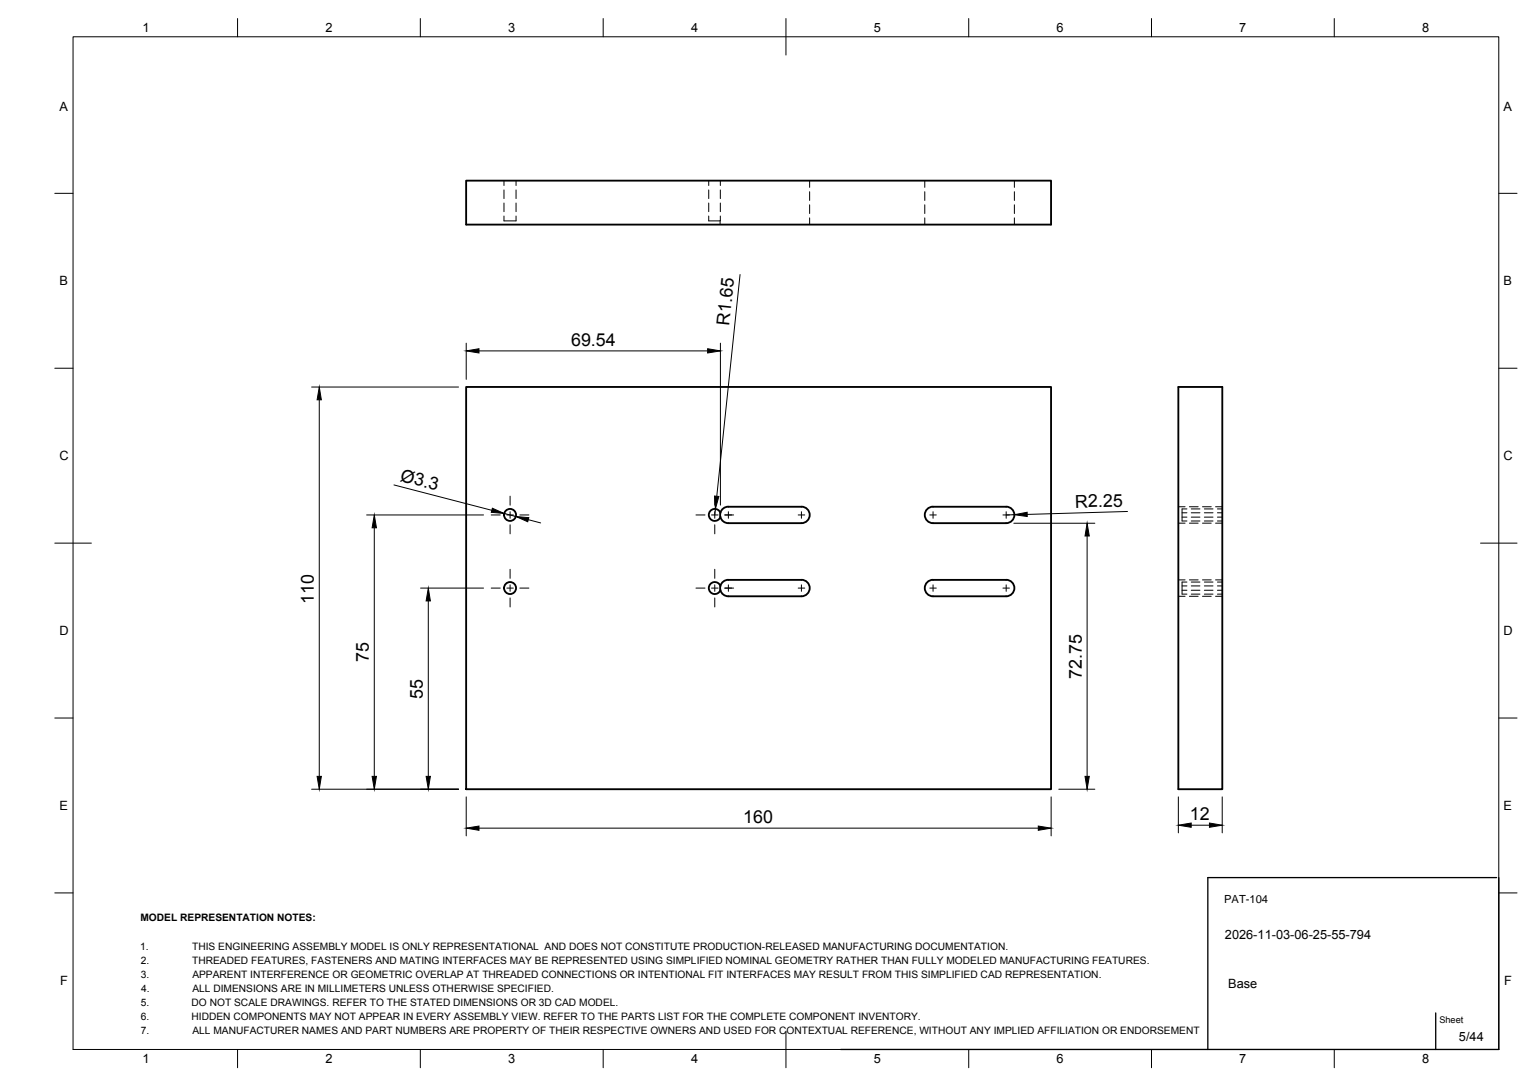
ISO-10303-21;
HEADER;
/* Generated by software containing ST-Developer
 * from STEP Tools, Inc. (www.steptools.com) 
 */

FILE_DESCRIPTION(
/* description */ ('Timing belt drive module 2 mm Pitch Timing 20T-40T'),

/* implementation_level */ '2;1');

FILE_NAME(
/* name */ 'Base.step',
/* time_stamp */ '2026-10-28T03:25:12-07:00',
/* author */ (''),
/* organization */ (''),
/* preprocessor_version */ 'ST-DEVELOPER v20.2',
/* originating_system */ 'Autodesk Translation Framework v15.17.0.0',
/* authorisation */ '');

FILE_SCHEMA (('AUTOMOTIVE_DESIGN { 1 0 10303 214 3 1 1 }'));
ENDSEC;

DATA;
#10=MECHANICAL_DESIGN_GEOMETRIC_PRESENTATION_REPRESENTATION('',(#524),#17830);
#438=SHAPE_REPRESENTATION_RELATIONSHIP('SRR','None',#18008,#481);
#481=ADVANCED_BREP_SHAPE_REPRESENTATION('',(#582),#17783);
#524=STYLED_ITEM('',(#18296),#582);
#582=MANIFOLD_SOLID_BREP('Body1',#8981);
#637=FACE_BOUND('',#1486,.T.);
#638=FACE_BOUND('',#1487,.T.);
#639=FACE_BOUND('',#1488,.T.);
#640=FACE_BOUND('',#1489,.T.);
#641=FACE_BOUND('',#1517,.T.);
#642=FACE_BOUND('',#1518,.T.);
#643=FACE_BOUND('',#1519,.T.);
#644=FACE_BOUND('',#1520,.T.);
#645=FACE_BOUND('',#1521,.T.);
#646=FACE_BOUND('',#1522,.T.);
#773=PLANE('',#9525);
#774=PLANE('',#9532);
#775=PLANE('',#9533);
#776=PLANE('',#9538);
#777=PLANE('',#9539);
#778=PLANE('',#9546);
#779=PLANE('',#9547);
#780=PLANE('',#9554);
#781=PLANE('',#9555);
#782=PLANE('',#9559);
#783=PLANE('',#9563);
#784=PLANE('',#9567);
#785=PLANE('',#9571);
#786=PLANE('',#9572);
#787=PLANE('',#9573);
#788=PLANE('',#9574);
#789=PLANE('',#9575);
#790=PLANE('',#9576);
#962=FACE_OUTER_BOUND('',#1483,.T.);
#963=FACE_OUTER_BOUND('',#1484,.T.);
#964=FACE_OUTER_BOUND('',#1485,.T.);
#965=FACE_OUTER_BOUND('',#1490,.T.);
#966=FACE_OUTER_BOUND('',#1491,.T.);
#967=FACE_OUTER_BOUND('',#1492,.T.);
#968=FACE_OUTER_BOUND('',#1493,.T.);
#969=FACE_OUTER_BOUND('',#1494,.T.);
#970=FACE_OUTER_BOUND('',#1495,.T.);
#971=FACE_OUTER_BOUND('',#1496,.T.);
#972=FACE_OUTER_BOUND('',#1497,.T.);
#973=FACE_OUTER_BOUND('',#1498,.T.);
#974=FACE_OUTER_BOUND('',#1499,.T.);
#975=FACE_OUTER_BOUND('',#1500,.T.);
#976=FACE_OUTER_BOUND('',#1501,.T.);
#977=FACE_OUTER_BOUND('',#1502,.T.);
#978=FACE_OUTER_BOUND('',#1503,.T.);
#979=FACE_OUTER_BOUND('',#1504,.T.);
#980=FACE_OUTER_BOUND('',#1505,.T.);
#981=FACE_OUTER_BOUND('',#1506,.T.);
#982=FACE_OUTER_BOUND('',#1507,.T.);
#983=FACE_OUTER_BOUND('',#1508,.T.);
#984=FACE_OUTER_BOUND('',#1509,.T.);
#985=FACE_OUTER_BOUND('',#1510,.T.);
#986=FACE_OUTER_BOUND('',#1511,.T.);
#987=FACE_OUTER_BOUND('',#1512,.T.);
#988=FACE_OUTER_BOUND('',#1513,.T.);
#989=FACE_OUTER_BOUND('',#1514,.T.);
#990=FACE_OUTER_BOUND('',#1515,.T.);
#991=FACE_OUTER_BOUND('',#1516,.T.);
#1483=EDGE_LOOP('',(#5773,#5774,#5775,#5776));
#1484=EDGE_LOOP('',(#5777,#5778,#5779,#5780));
#1485=EDGE_LOOP('',(#5781,#5782,#5783,#5784));
#1486=EDGE_LOOP('',(#5785,#5786,#5787,#5788));
#1487=EDGE_LOOP('',(#5789,#5790,#5791,#5792));
#1488=EDGE_LOOP('',(#5793,#5794,#5795,#5796));
#1489=EDGE_LOOP('',(#5797,#5798,#5799,#5800));
#1490=EDGE_LOOP('',(#5801,#5802,#5803,#5804));
#1491=EDGE_LOOP('',(#5805,#5806,#5807,#5808));
#1492=EDGE_LOOP('',(#5809,#5810,#5811,#5812));
#1493=EDGE_LOOP('',(#5813,#5814,#5815,#5816));
#1494=EDGE_LOOP('',(#5817,#5818,#5819,#5820));
#1495=EDGE_LOOP('',(#5821,#5822,#5823,#5824));
#1496=EDGE_LOOP('',(#5825,#5826,#5827,#5828,#5829,#5830,#5831,#5832));
#1497=EDGE_LOOP('',(#5833,#5834,#5835,#5836));
#1498=EDGE_LOOP('',(#5837,#5838,#5839,#5840));
#1499=EDGE_LOOP('',(#5841,#5842,#5843,#5844));
#1500=EDGE_LOOP('',(#5845,#5846,#5847,#5848,#5849,#5850,#5851,#5852));
#1501=EDGE_LOOP('',(#5853,#5854,#5855,#5856));
#1502=EDGE_LOOP('',(#5857,#5858,#5859,#5860));
#1503=EDGE_LOOP('',(#5861,#5862,#5863,#5864));
#1504=EDGE_LOOP('',(#5865,#5866,#5867,#5868));
#1505=EDGE_LOOP('',(#5869,#5870));
#1506=EDGE_LOOP('',(#5871,#5872,#5873,#5874));
#1507=EDGE_LOOP('',(#5875));
#1508=EDGE_LOOP('',(#5876,#5877,#5878,#5879));
#1509=EDGE_LOOP('',(#5880));
#1510=EDGE_LOOP('',(#5881,#5882,#5883,#5884));
#1511=EDGE_LOOP('',(#5885,#5886));
#1512=EDGE_LOOP('',(#5887,#5888,#5889,#5890));
#1513=EDGE_LOOP('',(#5891,#5892,#5893,#5894));
#1514=EDGE_LOOP('',(#5895,#5896,#5897,#5898));
#1515=EDGE_LOOP('',(#5899,#5900,#5901,#5902));
#1516=EDGE_LOOP('',(#5903,#5904,#5905,#5906));
#1517=EDGE_LOOP('',(#5907,#5908,#5909,#5910));
#1518=EDGE_LOOP('',(#5911,#5912,#5913,#5914));
#1519=EDGE_LOOP('',(#5915,#5916,#5917,#5918,#5919,#5920));
#1520=EDGE_LOOP('',(#5921,#5922,#5923,#5924,#5925,#5926));
#1521=EDGE_LOOP('',(#5927));
#1522=EDGE_LOOP('',(#5928));
#2140=CIRCLE('',#9520,0.225);
#2141=CIRCLE('',#9521,0.225);
#2142=CIRCLE('',#9523,0.225);
#2143=CIRCLE('',#9524,0.225);
#2144=CIRCLE('',#9526,0.225);
#2145=CIRCLE('',#9527,0.225);
#2146=CIRCLE('',#9528,0.225);
#2147=CIRCLE('',#9529,0.225);
#2148=CIRCLE('',#9530,0.225);
#2149=CIRCLE('',#9531,0.225);
#2150=CIRCLE('',#9535,0.225);
#2151=CIRCLE('',#9537,0.225);
#2152=CIRCLE('',#9541,0.225);
#2153=CIRCLE('',#9542,0.225);
#2154=CIRCLE('',#9543,0.225);
#2155=CIRCLE('',#9545,0.225);
#2156=CIRCLE('',#9549,0.225);
#2157=CIRCLE('',#9550,0.225);
#2158=CIRCLE('',#9551,0.225);
#2159=CIRCLE('',#9553,0.225);
#2160=CIRCLE('',#9557,0.165);
#2161=CIRCLE('',#9558,0.165);
#2162=CIRCLE('',#9561,0.165);
#2163=CIRCLE('',#9562,0.165);
#2164=CIRCLE('',#9565,0.165);
#2165=CIRCLE('',#9566,0.165);
#2166=CIRCLE('',#9569,0.165);
#2167=CIRCLE('',#9570,0.165);
#2790=LINE('',#13879,#3268);
#2791=LINE('',#13883,#3269);
#2792=LINE('',#13888,#3270);
#2793=LINE('',#13892,#3271);
#2794=LINE('',#13897,#3272);
#2795=LINE('',#13899,#3273);
#2796=LINE('',#13901,#3274);
#2797=LINE('',#13902,#3275);
#2798=LINE('',#13907,#3276);
#2799=LINE('',#13910,#3277);
#2800=LINE('',#13915,#3278);
#2801=LINE('',#13918,#3279);
#2802=LINE('',#13923,#3280);
#2803=LINE('',#13926,#3281);
#2804=LINE('',#13927,#3282);
#2805=LINE('',#13928,#3283);
#2806=LINE('',#13930,#3284);
#2807=LINE('',#13932,#3285);
#2808=LINE('',#13935,#3286);
#2809=LINE('',#13937,#3287);
#2810=LINE('',#13941,#3288);
#2811=LINE('',#13944,#3289);
#2812=LINE('',#13946,#3290);
#2813=LINE('',#13948,#3291);
#2814=LINE('',#13952,#3292);
#2815=LINE('',#13955,#3293);
#2816=LINE('',#13957,#3294);
#2817=LINE('',#13961,#3295);
#2818=LINE('',#13965,#3296);
#2819=LINE('',#13968,#3297);
#2820=LINE('',#13970,#3298);
#2821=LINE('',#13972,#3299);
#2822=LINE('',#13976,#3300);
#2823=LINE('',#13979,#3301);
#2824=LINE('',#13981,#3302);
#2825=LINE('',#13985,#3303);
#2826=LINE('',#13989,#3304);
#2827=LINE('',#13992,#3305);
#2828=LINE('',#13994,#3306);
#2829=LINE('',#13996,#3307);
#2830=LINE('',#14005,#3308);
#2831=LINE('',#14012,#3309);
#2832=LINE('',#14021,#3310);
#2833=LINE('',#14023,#3311);
#2834=LINE('',#14024,#3312);
#2835=LINE('',#14027,#3313);
#2836=LINE('',#14028,#3314);
#2837=LINE('',#14031,#3315);
#2838=LINE('',#14032,#3316);
#2839=LINE('',#14034,#3317);
#3268=VECTOR('',#10817,1.);
#3269=VECTOR('',#10820,1.);
#3270=VECTOR('',#10825,1.);
#3271=VECTOR('',#10828,1.);
#3272=VECTOR('',#10833,1.);
#3273=VECTOR('',#10834,1.);
#3274=VECTOR('',#10835,1.);
#3275=VECTOR('',#10836,1.);
#3276=VECTOR('',#10839,1.);
#3277=VECTOR('',#10842,1.);
#3278=VECTOR('',#10845,1.);
#3279=VECTOR('',#10848,1.);
#3280=VECTOR('',#10851,1.);
#3281=VECTOR('',#10854,1.);
#3282=VECTOR('',#10855,1.);
#3283=VECTOR('',#10856,1.);
#3284=VECTOR('',#10859,1.);
#3285=VECTOR('',#10862,1.);
#3286=VECTOR('',#10865,1.);
#3287=VECTOR('',#10866,1.);
#3288=VECTOR('',#10871,1.);
#3289=VECTOR('',#10874,1.);
#3290=VECTOR('',#10877,1.);
#3291=VECTOR('',#10880,1.);
#3292=VECTOR('',#10883,1.);
#3293=VECTOR('',#10886,1.);
#3294=VECTOR('',#10887,1.);
#3295=VECTOR('',#10890,1.);
#3296=VECTOR('',#10895,1.);
#3297=VECTOR('',#10898,1.);
#3298=VECTOR('',#10901,1.);
#3299=VECTOR('',#10904,1.);
#3300=VECTOR('',#10907,1.);
#3301=VECTOR('',#10910,1.);
#3302=VECTOR('',#10911,1.);
#3303=VECTOR('',#10914,1.);
#3304=VECTOR('',#10919,1.);
#3305=VECTOR('',#10922,1.);
#3306=VECTOR('',#10925,1.);
#3307=VECTOR('',#10928,1.);
#3308=VECTOR('',#10941,0.165);
#3309=VECTOR('',#10950,0.165);
#3310=VECTOR('',#10965,1.);
#3311=VECTOR('',#10966,1.);
#3312=VECTOR('',#10967,1.);
#3313=VECTOR('',#10970,1.);
#3314=VECTOR('',#10971,1.);
#3315=VECTOR('',#10974,1.);
#3316=VECTOR('',#10975,1.);
#3317=VECTOR('',#10978,1.);
#3746=VERTEX_POINT('',#13877);
#3747=VERTEX_POINT('',#13878);
#3748=VERTEX_POINT('',#13880);
#3749=VERTEX_POINT('',#13882);
#3750=VERTEX_POINT('',#13886);
#3751=VERTEX_POINT('',#13887);
#3752=VERTEX_POINT('',#13889);
#3753=VERTEX_POINT('',#13891);
#3754=VERTEX_POINT('',#13895);
#3755=VERTEX_POINT('',#13896);
#3756=VERTEX_POINT('',#13898);
#3757=VERTEX_POINT('',#13900);
#3758=VERTEX_POINT('',#13903);
#3759=VERTEX_POINT('',#13904);
#3760=VERTEX_POINT('',#13906);
#3761=VERTEX_POINT('',#13908);
#3762=VERTEX_POINT('',#13911);
#3763=VERTEX_POINT('',#13912);
#3764=VERTEX_POINT('',#13914);
#3765=VERTEX_POINT('',#13916);
#3766=VERTEX_POINT('',#13919);
#3767=VERTEX_POINT('',#13920);
#3768=VERTEX_POINT('',#13922);
#3769=VERTEX_POINT('',#13924);
#3770=VERTEX_POINT('',#13934);
#3771=VERTEX_POINT('',#13936);
#3772=VERTEX_POINT('',#13940);
#3773=VERTEX_POINT('',#13942);
#3774=VERTEX_POINT('',#13950);
#3775=VERTEX_POINT('',#13951);
#3776=VERTEX_POINT('',#13953);
#3777=VERTEX_POINT('',#13956);
#3778=VERTEX_POINT('',#13958);
#3779=VERTEX_POINT('',#13960);
#3780=VERTEX_POINT('',#13964);
#3781=VERTEX_POINT('',#13966);
#3782=VERTEX_POINT('',#13974);
#3783=VERTEX_POINT('',#13975);
#3784=VERTEX_POINT('',#13977);
#3785=VERTEX_POINT('',#13980);
#3786=VERTEX_POINT('',#13982);
#3787=VERTEX_POINT('',#13984);
#3788=VERTEX_POINT('',#13988);
#3789=VERTEX_POINT('',#13990);
#3790=VERTEX_POINT('',#14002);
#3791=VERTEX_POINT('',#14004);
#3792=VERTEX_POINT('',#14009);
#3793=VERTEX_POINT('',#14011);
#3794=VERTEX_POINT('',#14020);
#3795=VERTEX_POINT('',#14022);
#3796=VERTEX_POINT('',#14026);
#3797=VERTEX_POINT('',#14030);
#4569=EDGE_CURVE('',#3746,#3747,#2790,.T.);
#4570=EDGE_CURVE('',#3748,#3746,#2140,.T.);
#4571=EDGE_CURVE('',#3748,#3749,#2791,.T.);
#4572=EDGE_CURVE('',#3747,#3749,#2141,.T.);
#4573=EDGE_CURVE('',#3750,#3751,#2792,.T.);
#4574=EDGE_CURVE('',#3752,#3751,#2142,.T.);
#4575=EDGE_CURVE('',#3753,#3752,#2793,.T.);
#4576=EDGE_CURVE('',#3750,#3753,#2143,.T.);
#4577=EDGE_CURVE('',#3754,#3755,#2794,.T.);
#4578=EDGE_CURVE('',#3756,#3754,#2795,.T.);
#4579=EDGE_CURVE('',#3757,#3756,#2796,.T.);
#4580=EDGE_CURVE('',#3755,#3757,#2797,.T.);
#4581=EDGE_CURVE('',#3758,#3759,#2144,.T.);
#4582=EDGE_CURVE('',#3759,#3760,#2798,.T.);
#4583=EDGE_CURVE('',#3760,#3761,#2145,.T.);
#4584=EDGE_CURVE('',#3761,#3758,#2799,.T.);
#4585=EDGE_CURVE('',#3762,#3763,#2146,.T.);
#4586=EDGE_CURVE('',#3763,#3764,#2800,.T.);
#4587=EDGE_CURVE('',#3764,#3765,#2147,.T.);
#4588=EDGE_CURVE('',#3765,#3762,#2801,.T.);
#4589=EDGE_CURVE('',#3766,#3767,#2148,.T.);
#4590=EDGE_CURVE('',#3767,#3768,#2802,.T.);
#4591=EDGE_CURVE('',#3768,#3769,#2149,.T.);
#4592=EDGE_CURVE('',#3769,#3766,#2803,.T.);
#4593=EDGE_CURVE('',#3746,#3750,#2804,.T.);
#4594=EDGE_CURVE('',#3753,#3748,#2805,.T.);
#4595=EDGE_CURVE('',#3749,#3752,#2806,.T.);
#4596=EDGE_CURVE('',#3751,#3747,#2807,.T.);
#4597=EDGE_CURVE('',#3759,#3770,#2808,.T.);
#4598=EDGE_CURVE('',#3758,#3771,#2809,.T.);
#4599=EDGE_CURVE('',#3770,#3771,#2150,.T.);
#4600=EDGE_CURVE('',#3760,#3772,#2810,.T.);
#4601=EDGE_CURVE('',#3773,#3772,#2151,.T.);
#4602=EDGE_CURVE('',#3761,#3773,#2811,.T.);
#4603=EDGE_CURVE('',#3771,#3773,#2812,.T.);
#4604=EDGE_CURVE('',#3772,#3770,#2813,.T.);
#4605=EDGE_CURVE('',#3774,#3775,#2814,.T.);
#4606=EDGE_CURVE('',#3776,#3774,#2152,.T.);
#4607=EDGE_CURVE('',#3767,#3776,#2815,.T.);
#4608=EDGE_CURVE('',#3766,#3777,#2816,.T.);
#4609=EDGE_CURVE('',#3778,#3777,#2153,.T.);
#4610=EDGE_CURVE('',#3779,#3778,#2817,.T.);
#4611=EDGE_CURVE('',#3775,#3779,#2154,.T.);
#4612=EDGE_CURVE('',#3768,#3780,#2818,.T.);
#4613=EDGE_CURVE('',#3781,#3780,#2155,.T.);
#4614=EDGE_CURVE('',#3769,#3781,#2819,.T.);
#4615=EDGE_CURVE('',#3777,#3781,#2820,.T.);
#4616=EDGE_CURVE('',#3780,#3776,#2821,.T.);
#4617=EDGE_CURVE('',#3782,#3783,#2822,.T.);
#4618=EDGE_CURVE('',#3784,#3782,#2156,.T.);
#4619=EDGE_CURVE('',#3763,#3784,#2823,.T.);
#4620=EDGE_CURVE('',#3762,#3785,#2824,.T.);
#4621=EDGE_CURVE('',#3786,#3785,#2157,.T.);
#4622=EDGE_CURVE('',#3787,#3786,#2825,.T.);
#4623=EDGE_CURVE('',#3783,#3787,#2158,.T.);
#4624=EDGE_CURVE('',#3764,#3788,#2826,.T.);
#4625=EDGE_CURVE('',#3789,#3788,#2159,.T.);
#4626=EDGE_CURVE('',#3765,#3789,#2827,.T.);
#4627=EDGE_CURVE('',#3785,#3789,#2828,.T.);
#4628=EDGE_CURVE('',#3788,#3784,#2829,.T.);
#4629=EDGE_CURVE('',#3782,#3786,#2160,.T.);
#4630=EDGE_CURVE('',#3787,#3783,#2161,.T.);
#4631=EDGE_CURVE('',#3790,#3790,#2162,.T.);
#4632=EDGE_CURVE('',#3790,#3791,#2830,.T.);
#4633=EDGE_CURVE('',#3791,#3791,#2163,.T.);
#4634=EDGE_CURVE('',#3792,#3792,#2164,.T.);
#4635=EDGE_CURVE('',#3792,#3793,#2831,.T.);
#4636=EDGE_CURVE('',#3793,#3793,#2165,.T.);
#4637=EDGE_CURVE('',#3774,#3778,#2166,.T.);
#4638=EDGE_CURVE('',#3779,#3775,#2167,.T.);
#4639=EDGE_CURVE('',#3754,#3794,#2832,.T.);
#4640=EDGE_CURVE('',#3795,#3794,#2833,.T.);
#4641=EDGE_CURVE('',#3756,#3795,#2834,.T.);
#4642=EDGE_CURVE('',#3796,#3795,#2835,.T.);
#4643=EDGE_CURVE('',#3757,#3796,#2836,.T.);
#4644=EDGE_CURVE('',#3797,#3796,#2837,.T.);
#4645=EDGE_CURVE('',#3755,#3797,#2838,.T.);
#4646=EDGE_CURVE('',#3794,#3797,#2839,.T.);
#5773=ORIENTED_EDGE('',*,*,#4569,.F.);
#5774=ORIENTED_EDGE('',*,*,#4570,.F.);
#5775=ORIENTED_EDGE('',*,*,#4571,.T.);
#5776=ORIENTED_EDGE('',*,*,#4572,.F.);
#5777=ORIENTED_EDGE('',*,*,#4573,.T.);
#5778=ORIENTED_EDGE('',*,*,#4574,.F.);
#5779=ORIENTED_EDGE('',*,*,#4575,.F.);
#5780=ORIENTED_EDGE('',*,*,#4576,.F.);
#5781=ORIENTED_EDGE('',*,*,#4577,.F.);
#5782=ORIENTED_EDGE('',*,*,#4578,.F.);
#5783=ORIENTED_EDGE('',*,*,#4579,.F.);
#5784=ORIENTED_EDGE('',*,*,#4580,.F.);
#5785=ORIENTED_EDGE('',*,*,#4581,.T.);
#5786=ORIENTED_EDGE('',*,*,#4582,.T.);
#5787=ORIENTED_EDGE('',*,*,#4583,.T.);
#5788=ORIENTED_EDGE('',*,*,#4584,.T.);
#5789=ORIENTED_EDGE('',*,*,#4585,.T.);
#5790=ORIENTED_EDGE('',*,*,#4586,.T.);
#5791=ORIENTED_EDGE('',*,*,#4587,.T.);
#5792=ORIENTED_EDGE('',*,*,#4588,.T.);
#5793=ORIENTED_EDGE('',*,*,#4589,.T.);
#5794=ORIENTED_EDGE('',*,*,#4590,.T.);
#5795=ORIENTED_EDGE('',*,*,#4591,.T.);
#5796=ORIENTED_EDGE('',*,*,#4592,.T.);
#5797=ORIENTED_EDGE('',*,*,#4570,.T.);
#5798=ORIENTED_EDGE('',*,*,#4593,.T.);
#5799=ORIENTED_EDGE('',*,*,#4576,.T.);
#5800=ORIENTED_EDGE('',*,*,#4594,.T.);
#5801=ORIENTED_EDGE('',*,*,#4595,.F.);
#5802=ORIENTED_EDGE('',*,*,#4571,.F.);
#5803=ORIENTED_EDGE('',*,*,#4594,.F.);
#5804=ORIENTED_EDGE('',*,*,#4575,.T.);
#5805=ORIENTED_EDGE('',*,*,#4593,.F.);
#5806=ORIENTED_EDGE('',*,*,#4569,.T.);
#5807=ORIENTED_EDGE('',*,*,#4596,.F.);
#5808=ORIENTED_EDGE('',*,*,#4573,.F.);
#5809=ORIENTED_EDGE('',*,*,#4597,.F.);
#5810=ORIENTED_EDGE('',*,*,#4581,.F.);
#5811=ORIENTED_EDGE('',*,*,#4598,.T.);
#5812=ORIENTED_EDGE('',*,*,#4599,.F.);
#5813=ORIENTED_EDGE('',*,*,#4600,.T.);
#5814=ORIENTED_EDGE('',*,*,#4601,.F.);
#5815=ORIENTED_EDGE('',*,*,#4602,.F.);
#5816=ORIENTED_EDGE('',*,*,#4583,.F.);
#5817=ORIENTED_EDGE('',*,*,#4603,.F.);
#5818=ORIENTED_EDGE('',*,*,#4598,.F.);
#5819=ORIENTED_EDGE('',*,*,#4584,.F.);
#5820=ORIENTED_EDGE('',*,*,#4602,.T.);
#5821=ORIENTED_EDGE('',*,*,#4582,.F.);
#5822=ORIENTED_EDGE('',*,*,#4597,.T.);
#5823=ORIENTED_EDGE('',*,*,#4604,.F.);
#5824=ORIENTED_EDGE('',*,*,#4600,.F.);
#5825=ORIENTED_EDGE('',*,*,#4605,.F.);
#5826=ORIENTED_EDGE('',*,*,#4606,.F.);
#5827=ORIENTED_EDGE('',*,*,#4607,.F.);
#5828=ORIENTED_EDGE('',*,*,#4589,.F.);
#5829=ORIENTED_EDGE('',*,*,#4608,.T.);
#5830=ORIENTED_EDGE('',*,*,#4609,.F.);
#5831=ORIENTED_EDGE('',*,*,#4610,.F.);
#5832=ORIENTED_EDGE('',*,*,#4611,.F.);
#5833=ORIENTED_EDGE('',*,*,#4612,.T.);
#5834=ORIENTED_EDGE('',*,*,#4613,.F.);
#5835=ORIENTED_EDGE('',*,*,#4614,.F.);
#5836=ORIENTED_EDGE('',*,*,#4591,.F.);
#5837=ORIENTED_EDGE('',*,*,#4615,.F.);
#5838=ORIENTED_EDGE('',*,*,#4608,.F.);
#5839=ORIENTED_EDGE('',*,*,#4592,.F.);
#5840=ORIENTED_EDGE('',*,*,#4614,.T.);
#5841=ORIENTED_EDGE('',*,*,#4590,.F.);
#5842=ORIENTED_EDGE('',*,*,#4607,.T.);
#5843=ORIENTED_EDGE('',*,*,#4616,.F.);
#5844=ORIENTED_EDGE('',*,*,#4612,.F.);
#5845=ORIENTED_EDGE('',*,*,#4617,.F.);
#5846=ORIENTED_EDGE('',*,*,#4618,.F.);
#5847=ORIENTED_EDGE('',*,*,#4619,.F.);
#5848=ORIENTED_EDGE('',*,*,#4585,.F.);
#5849=ORIENTED_EDGE('',*,*,#4620,.T.);
#5850=ORIENTED_EDGE('',*,*,#4621,.F.);
#5851=ORIENTED_EDGE('',*,*,#4622,.F.);
#5852=ORIENTED_EDGE('',*,*,#4623,.F.);
#5853=ORIENTED_EDGE('',*,*,#4624,.T.);
#5854=ORIENTED_EDGE('',*,*,#4625,.F.);
#5855=ORIENTED_EDGE('',*,*,#4626,.F.);
#5856=ORIENTED_EDGE('',*,*,#4587,.F.);
#5857=ORIENTED_EDGE('',*,*,#4627,.F.);
#5858=ORIENTED_EDGE('',*,*,#4620,.F.);
#5859=ORIENTED_EDGE('',*,*,#4588,.F.);
#5860=ORIENTED_EDGE('',*,*,#4626,.T.);
#5861=ORIENTED_EDGE('',*,*,#4586,.F.);
#5862=ORIENTED_EDGE('',*,*,#4619,.T.);
#5863=ORIENTED_EDGE('',*,*,#4628,.F.);
#5864=ORIENTED_EDGE('',*,*,#4624,.F.);
#5865=ORIENTED_EDGE('',*,*,#4622,.T.);
#5866=ORIENTED_EDGE('',*,*,#4629,.F.);
#5867=ORIENTED_EDGE('',*,*,#4617,.T.);
#5868=ORIENTED_EDGE('',*,*,#4630,.F.);
#5869=ORIENTED_EDGE('',*,*,#4623,.T.);
#5870=ORIENTED_EDGE('',*,*,#4630,.T.);
#5871=ORIENTED_EDGE('',*,*,#4631,.F.);
#5872=ORIENTED_EDGE('',*,*,#4632,.T.);
#5873=ORIENTED_EDGE('',*,*,#4633,.F.);
#5874=ORIENTED_EDGE('',*,*,#4632,.F.);
#5875=ORIENTED_EDGE('',*,*,#4631,.T.);
#5876=ORIENTED_EDGE('',*,*,#4634,.F.);
#5877=ORIENTED_EDGE('',*,*,#4635,.T.);
#5878=ORIENTED_EDGE('',*,*,#4636,.F.);
#5879=ORIENTED_EDGE('',*,*,#4635,.F.);
#5880=ORIENTED_EDGE('',*,*,#4634,.T.);
#5881=ORIENTED_EDGE('',*,*,#4610,.T.);
#5882=ORIENTED_EDGE('',*,*,#4637,.F.);
#5883=ORIENTED_EDGE('',*,*,#4605,.T.);
#5884=ORIENTED_EDGE('',*,*,#4638,.F.);
#5885=ORIENTED_EDGE('',*,*,#4611,.T.);
#5886=ORIENTED_EDGE('',*,*,#4638,.T.);
#5887=ORIENTED_EDGE('',*,*,#4578,.T.);
#5888=ORIENTED_EDGE('',*,*,#4639,.T.);
#5889=ORIENTED_EDGE('',*,*,#4640,.F.);
#5890=ORIENTED_EDGE('',*,*,#4641,.F.);
#5891=ORIENTED_EDGE('',*,*,#4579,.T.);
#5892=ORIENTED_EDGE('',*,*,#4641,.T.);
#5893=ORIENTED_EDGE('',*,*,#4642,.F.);
#5894=ORIENTED_EDGE('',*,*,#4643,.F.);
#5895=ORIENTED_EDGE('',*,*,#4580,.T.);
#5896=ORIENTED_EDGE('',*,*,#4643,.T.);
#5897=ORIENTED_EDGE('',*,*,#4644,.F.);
#5898=ORIENTED_EDGE('',*,*,#4645,.F.);
#5899=ORIENTED_EDGE('',*,*,#4577,.T.);
#5900=ORIENTED_EDGE('',*,*,#4645,.T.);
#5901=ORIENTED_EDGE('',*,*,#4646,.F.);
#5902=ORIENTED_EDGE('',*,*,#4639,.F.);
#5903=ORIENTED_EDGE('',*,*,#4646,.T.);
#5904=ORIENTED_EDGE('',*,*,#4644,.T.);
#5905=ORIENTED_EDGE('',*,*,#4642,.T.);
#5906=ORIENTED_EDGE('',*,*,#4640,.T.);
#5907=ORIENTED_EDGE('',*,*,#4572,.T.);
#5908=ORIENTED_EDGE('',*,*,#4595,.T.);
#5909=ORIENTED_EDGE('',*,*,#4574,.T.);
#5910=ORIENTED_EDGE('',*,*,#4596,.T.);
#5911=ORIENTED_EDGE('',*,*,#4599,.T.);
#5912=ORIENTED_EDGE('',*,*,#4603,.T.);
#5913=ORIENTED_EDGE('',*,*,#4601,.T.);
#5914=ORIENTED_EDGE('',*,*,#4604,.T.);
#5915=ORIENTED_EDGE('',*,*,#4609,.T.);
#5916=ORIENTED_EDGE('',*,*,#4615,.T.);
#5917=ORIENTED_EDGE('',*,*,#4613,.T.);
#5918=ORIENTED_EDGE('',*,*,#4616,.T.);
#5919=ORIENTED_EDGE('',*,*,#4606,.T.);
#5920=ORIENTED_EDGE('',*,*,#4637,.T.);
#5921=ORIENTED_EDGE('',*,*,#4621,.T.);
#5922=ORIENTED_EDGE('',*,*,#4627,.T.);
#5923=ORIENTED_EDGE('',*,*,#4625,.T.);
#5924=ORIENTED_EDGE('',*,*,#4628,.T.);
#5925=ORIENTED_EDGE('',*,*,#4618,.T.);
#5926=ORIENTED_EDGE('',*,*,#4629,.T.);
#5927=ORIENTED_EDGE('',*,*,#4633,.T.);
#5928=ORIENTED_EDGE('',*,*,#4636,.T.);
#8181=CYLINDRICAL_SURFACE('',#9519,0.225);
#8182=CYLINDRICAL_SURFACE('',#9522,0.225);
#8183=CYLINDRICAL_SURFACE('',#9534,0.225);
#8184=CYLINDRICAL_SURFACE('',#9536,0.225);
#8185=CYLINDRICAL_SURFACE('',#9540,0.225);
#8186=CYLINDRICAL_SURFACE('',#9544,0.225);
#8187=CYLINDRICAL_SURFACE('',#9548,0.225);
#8188=CYLINDRICAL_SURFACE('',#9552,0.225);
#8189=CYLINDRICAL_SURFACE('',#9556,0.165);
#8190=CYLINDRICAL_SURFACE('',#9560,0.165);
#8191=CYLINDRICAL_SURFACE('',#9564,0.165);
#8192=CYLINDRICAL_SURFACE('',#9568,0.165);
#8460=ADVANCED_FACE('',(#962),#8181,.F.);
#8461=ADVANCED_FACE('',(#963),#8182,.F.);
#8462=ADVANCED_FACE('',(#964,#637,#638,#639,#640),#773,.F.);
#8463=ADVANCED_FACE('',(#965),#774,.F.);
#8464=ADVANCED_FACE('',(#966),#775,.F.);
#8465=ADVANCED_FACE('',(#967),#8183,.F.);
#8466=ADVANCED_FACE('',(#968),#8184,.F.);
#8467=ADVANCED_FACE('',(#969),#776,.F.);
#8468=ADVANCED_FACE('',(#970),#777,.F.);
#8469=ADVANCED_FACE('',(#971),#8185,.F.);
#8470=ADVANCED_FACE('',(#972),#8186,.F.);
#8471=ADVANCED_FACE('',(#973),#778,.F.);
#8472=ADVANCED_FACE('',(#974),#779,.F.);
#8473=ADVANCED_FACE('',(#975),#8187,.F.);
#8474=ADVANCED_FACE('',(#976),#8188,.F.);
#8475=ADVANCED_FACE('',(#977),#780,.F.);
#8476=ADVANCED_FACE('',(#978),#781,.F.);
#8477=ADVANCED_FACE('',(#979),#8189,.F.);
#8478=ADVANCED_FACE('',(#980),#782,.T.);
#8479=ADVANCED_FACE('',(#981),#8190,.F.);
#8480=ADVANCED_FACE('',(#982),#783,.T.);
#8481=ADVANCED_FACE('',(#983),#8191,.F.);
#8482=ADVANCED_FACE('',(#984),#784,.T.);
#8483=ADVANCED_FACE('',(#985),#8192,.F.);
#8484=ADVANCED_FACE('',(#986),#785,.T.);
#8485=ADVANCED_FACE('',(#987),#786,.T.);
#8486=ADVANCED_FACE('',(#988),#787,.T.);
#8487=ADVANCED_FACE('',(#989),#788,.T.);
#8488=ADVANCED_FACE('',(#990),#789,.T.);
#8489=ADVANCED_FACE('',(#991,#641,#642,#643,#644,#645,#646),#790,.T.);
#8981=CLOSED_SHELL('',(#8460,#8461,#8462,#8463,#8464,#8465,#8466,#8467,
#8468,#8469,#8470,#8471,#8472,#8473,#8474,#8475,#8476,#8477,#8478,#8479,
#8480,#8481,#8482,#8483,#8484,#8485,#8486,#8487,#8488,#8489));
#9518=AXIS2_PLACEMENT_3D('',#13875,#10813,#10814);
#9519=AXIS2_PLACEMENT_3D('',#13876,#10815,#10816);
#9520=AXIS2_PLACEMENT_3D('',#13881,#10818,#10819);
#9521=AXIS2_PLACEMENT_3D('',#13884,#10821,#10822);
#9522=AXIS2_PLACEMENT_3D('',#13885,#10823,#10824);
#9523=AXIS2_PLACEMENT_3D('',#13890,#10826,#10827);
#9524=AXIS2_PLACEMENT_3D('',#13893,#10829,#10830);
#9525=AXIS2_PLACEMENT_3D('',#13894,#10831,#10832);
#9526=AXIS2_PLACEMENT_3D('',#13905,#10837,#10838);
#9527=AXIS2_PLACEMENT_3D('',#13909,#10840,#10841);
#9528=AXIS2_PLACEMENT_3D('',#13913,#10843,#10844);
#9529=AXIS2_PLACEMENT_3D('',#13917,#10846,#10847);
#9530=AXIS2_PLACEMENT_3D('',#13921,#10849,#10850);
#9531=AXIS2_PLACEMENT_3D('',#13925,#10852,#10853);
#9532=AXIS2_PLACEMENT_3D('',#13929,#10857,#10858);
#9533=AXIS2_PLACEMENT_3D('',#13931,#10860,#10861);
#9534=AXIS2_PLACEMENT_3D('',#13933,#10863,#10864);
#9535=AXIS2_PLACEMENT_3D('',#13938,#10867,#10868);
#9536=AXIS2_PLACEMENT_3D('',#13939,#10869,#10870);
#9537=AXIS2_PLACEMENT_3D('',#13943,#10872,#10873);
#9538=AXIS2_PLACEMENT_3D('',#13945,#10875,#10876);
#9539=AXIS2_PLACEMENT_3D('',#13947,#10878,#10879);
#9540=AXIS2_PLACEMENT_3D('',#13949,#10881,#10882);
#9541=AXIS2_PLACEMENT_3D('',#13954,#10884,#10885);
#9542=AXIS2_PLACEMENT_3D('',#13959,#10888,#10889);
#9543=AXIS2_PLACEMENT_3D('',#13962,#10891,#10892);
#9544=AXIS2_PLACEMENT_3D('',#13963,#10893,#10894);
#9545=AXIS2_PLACEMENT_3D('',#13967,#10896,#10897);
#9546=AXIS2_PLACEMENT_3D('',#13969,#10899,#10900);
#9547=AXIS2_PLACEMENT_3D('',#13971,#10902,#10903);
#9548=AXIS2_PLACEMENT_3D('',#13973,#10905,#10906);
#9549=AXIS2_PLACEMENT_3D('',#13978,#10908,#10909);
#9550=AXIS2_PLACEMENT_3D('',#13983,#10912,#10913);
#9551=AXIS2_PLACEMENT_3D('',#13986,#10915,#10916);
#9552=AXIS2_PLACEMENT_3D('',#13987,#10917,#10918);
#9553=AXIS2_PLACEMENT_3D('',#13991,#10920,#10921);
#9554=AXIS2_PLACEMENT_3D('',#13993,#10923,#10924);
#9555=AXIS2_PLACEMENT_3D('',#13995,#10926,#10927);
#9556=AXIS2_PLACEMENT_3D('',#13997,#10929,#10930);
#9557=AXIS2_PLACEMENT_3D('',#13998,#10931,#10932);
#9558=AXIS2_PLACEMENT_3D('',#13999,#10933,#10934);
#9559=AXIS2_PLACEMENT_3D('',#14000,#10935,#10936);
#9560=AXIS2_PLACEMENT_3D('',#14001,#10937,#10938);
#9561=AXIS2_PLACEMENT_3D('',#14003,#10939,#10940);
#9562=AXIS2_PLACEMENT_3D('',#14006,#10942,#10943);
#9563=AXIS2_PLACEMENT_3D('',#14007,#10944,#10945);
#9564=AXIS2_PLACEMENT_3D('',#14008,#10946,#10947);
#9565=AXIS2_PLACEMENT_3D('',#14010,#10948,#10949);
#9566=AXIS2_PLACEMENT_3D('',#14013,#10951,#10952);
#9567=AXIS2_PLACEMENT_3D('',#14014,#10953,#10954);
#9568=AXIS2_PLACEMENT_3D('',#14015,#10955,#10956);
#9569=AXIS2_PLACEMENT_3D('',#14016,#10957,#10958);
#9570=AXIS2_PLACEMENT_3D('',#14017,#10959,#10960);
#9571=AXIS2_PLACEMENT_3D('',#14018,#10961,#10962);
#9572=AXIS2_PLACEMENT_3D('',#14019,#10963,#10964);
#9573=AXIS2_PLACEMENT_3D('',#14025,#10968,#10969);
#9574=AXIS2_PLACEMENT_3D('',#14029,#10972,#10973);
#9575=AXIS2_PLACEMENT_3D('',#14033,#10976,#10977);
#9576=AXIS2_PLACEMENT_3D('',#14035,#10979,#10980);
#10813=DIRECTION('axis',(0.,0.,1.));
#10814=DIRECTION('refdir',(1.,0.,0.));
#10815=DIRECTION('center_axis',(0.,0.,1.));
#10816=DIRECTION('ref_axis',(-1.,-1.22464679914735E-16,0.));
#10817=DIRECTION('',(0.,0.,1.));
#10818=DIRECTION('center_axis',(0.,0.,1.));
#10819=DIRECTION('ref_axis',(1.,0.,0.));
#10820=DIRECTION('',(0.,0.,1.));
#10821=DIRECTION('center_axis',(0.,0.,-1.));
#10822=DIRECTION('ref_axis',(1.,0.,0.));
#10823=DIRECTION('center_axis',(0.,0.,1.));
#10824=DIRECTION('ref_axis',(1.,0.,0.));
#10825=DIRECTION('',(0.,0.,1.));
#10826=DIRECTION('center_axis',(0.,0.,-1.));
#10827=DIRECTION('ref_axis',(1.,0.,0.));
#10828=DIRECTION('',(0.,0.,1.));
#10829=DIRECTION('center_axis',(0.,0.,1.));
#10830=DIRECTION('ref_axis',(1.,0.,0.));
#10831=DIRECTION('center_axis',(0.,0.,1.));
#10832=DIRECTION('ref_axis',(1.,0.,0.));
#10833=DIRECTION('',(0.,-1.,0.));
#10834=DIRECTION('',(-1.,0.,0.));
#10835=DIRECTION('',(0.,1.,0.));
#10836=DIRECTION('',(1.,0.,0.));
#10837=DIRECTION('center_axis',(0.,0.,1.));
#10838=DIRECTION('ref_axis',(1.,0.,0.));
#10839=DIRECTION('',(1.,0.,0.));
#10840=DIRECTION('center_axis',(0.,0.,1.));
#10841=DIRECTION('ref_axis',(1.,0.,0.));
#10842=DIRECTION('',(-1.,0.,0.));
#10843=DIRECTION('center_axis',(0.,0.,1.));
#10844=DIRECTION('ref_axis',(1.,0.,0.));
#10845=DIRECTION('',(1.,0.,0.));
#10846=DIRECTION('center_axis',(0.,0.,1.));
#10847=DIRECTION('ref_axis',(1.,0.,0.));
#10848=DIRECTION('',(-1.,0.,0.));
#10849=DIRECTION('center_axis',(0.,0.,1.));
#10850=DIRECTION('ref_axis',(1.,0.,0.));
#10851=DIRECTION('',(1.,0.,0.));
#10852=DIRECTION('center_axis',(0.,0.,1.));
#10853=DIRECTION('ref_axis',(1.,0.,0.));
#10854=DIRECTION('',(-1.,0.,0.));
#10855=DIRECTION('',(1.,0.,0.));
#10856=DIRECTION('',(-1.,0.,0.));
#10857=DIRECTION('center_axis',(0.,1.,0.));
#10858=DIRECTION('ref_axis',(-1.,0.,0.));
#10859=DIRECTION('',(1.,0.,0.));
#10860=DIRECTION('center_axis',(0.,-1.,0.));
#10861=DIRECTION('ref_axis',(1.,0.,0.));
#10862=DIRECTION('',(-1.,0.,0.));
#10863=DIRECTION('center_axis',(0.,0.,1.));
#10864=DIRECTION('ref_axis',(-1.,-1.22464679914735E-16,0.));
#10865=DIRECTION('',(0.,0.,1.));
#10866=DIRECTION('',(0.,0.,1.));
#10867=DIRECTION('center_axis',(0.,0.,-1.));
#10868=DIRECTION('ref_axis',(1.,0.,0.));
#10869=DIRECTION('center_axis',(0.,0.,1.));
#10870=DIRECTION('ref_axis',(1.,0.,0.));
#10871=DIRECTION('',(0.,0.,1.));
#10872=DIRECTION('center_axis',(0.,0.,-1.));
#10873=DIRECTION('ref_axis',(1.,0.,0.));
#10874=DIRECTION('',(0.,0.,1.));
#10875=DIRECTION('center_axis',(0.,1.,0.));
#10876=DIRECTION('ref_axis',(-1.,0.,0.));
#10877=DIRECTION('',(1.,0.,0.));
#10878=DIRECTION('center_axis',(0.,-1.,0.));
#10879=DIRECTION('ref_axis',(1.,0.,0.));
#10880=DIRECTION('',(-1.,0.,0.));
#10881=DIRECTION('center_axis',(0.,0.,1.));
#10882=DIRECTION('ref_axis',(-1.,-1.22464679914735E-16,0.));
#10883=DIRECTION('',(0.,0.,-1.));
#10884=DIRECTION('center_axis',(0.,0.,-1.));
#10885=DIRECTION('ref_axis',(1.,0.,0.));
#10886=DIRECTION('',(0.,0.,1.));
#10887=DIRECTION('',(0.,0.,1.));
#10888=DIRECTION('center_axis',(0.,0.,-1.));
#10889=DIRECTION('ref_axis',(1.,0.,0.));
#10890=DIRECTION('',(0.,0.,1.));
#10891=DIRECTION('center_axis',(0.,0.,-1.));
#10892=DIRECTION('ref_axis',(1.,0.,0.));
#10893=DIRECTION('center_axis',(0.,0.,1.));
#10894=DIRECTION('ref_axis',(1.,0.,0.));
#10895=DIRECTION('',(0.,0.,1.));
#10896=DIRECTION('center_axis',(0.,0.,-1.));
#10897=DIRECTION('ref_axis',(1.,0.,0.));
#10898=DIRECTION('',(0.,0.,1.));
#10899=DIRECTION('center_axis',(0.,1.,0.));
#10900=DIRECTION('ref_axis',(-1.,0.,0.));
#10901=DIRECTION('',(1.,0.,0.));
#10902=DIRECTION('center_axis',(0.,-1.,0.));
#10903=DIRECTION('ref_axis',(1.,0.,0.));
#10904=DIRECTION('',(-1.,0.,0.));
#10905=DIRECTION('center_axis',(0.,0.,1.));
#10906=DIRECTION('ref_axis',(-1.,-1.22464679914735E-16,0.));
#10907=DIRECTION('',(0.,0.,-1.));
#10908=DIRECTION('center_axis',(0.,0.,-1.));
#10909=DIRECTION('ref_axis',(1.,0.,0.));
#10910=DIRECTION('',(0.,0.,1.));
#10911=DIRECTION('',(0.,0.,1.));
#10912=DIRECTION('center_axis',(0.,0.,-1.));
#10913=DIRECTION('ref_axis',(1.,0.,0.));
#10914=DIRECTION('',(0.,0.,1.));
#10915=DIRECTION('center_axis',(0.,0.,-1.));
#10916=DIRECTION('ref_axis',(1.,0.,0.));
#10917=DIRECTION('center_axis',(0.,0.,1.));
#10918=DIRECTION('ref_axis',(1.,0.,0.));
#10919=DIRECTION('',(0.,0.,1.));
#10920=DIRECTION('center_axis',(0.,0.,-1.));
#10921=DIRECTION('ref_axis',(1.,0.,0.));
#10922=DIRECTION('',(0.,0.,1.));
#10923=DIRECTION('center_axis',(0.,1.,0.));
#10924=DIRECTION('ref_axis',(-1.,0.,0.));
#10925=DIRECTION('',(1.,0.,0.));
#10926=DIRECTION('center_axis',(0.,-1.,0.));
#10927=DIRECTION('ref_axis',(1.,0.,0.));
#10928=DIRECTION('',(-1.,0.,0.));
#10929=DIRECTION('center_axis',(0.,0.,1.));
#10930=DIRECTION('ref_axis',(-1.,5.66553889764798E-16,0.));
#10931=DIRECTION('center_axis',(0.,0.,-1.));
#10932=DIRECTION('ref_axis',(1.,0.,0.));
#10933=DIRECTION('center_axis',(0.,0.,1.));
#10934=DIRECTION('ref_axis',(1.,0.,0.));
#10935=DIRECTION('center_axis',(0.,0.,1.));
#10936=DIRECTION('ref_axis',(1.,0.,0.));
#10937=DIRECTION('center_axis',(0.,0.,1.));
#10938=DIRECTION('ref_axis',(1.,0.,0.));
#10939=DIRECTION('center_axis',(0.,0.,1.));
#10940=DIRECTION('ref_axis',(1.,0.,0.));
#10941=DIRECTION('',(0.,0.,1.));
#10942=DIRECTION('center_axis',(0.,0.,-1.));
#10943=DIRECTION('ref_axis',(1.,0.,0.));
#10944=DIRECTION('center_axis',(0.,0.,1.));
#10945=DIRECTION('ref_axis',(1.,0.,0.));
#10946=DIRECTION('center_axis',(0.,0.,1.));
#10947=DIRECTION('ref_axis',(1.,0.,0.));
#10948=DIRECTION('center_axis',(0.,0.,1.));
#10949=DIRECTION('ref_axis',(1.,0.,0.));
#10950=DIRECTION('',(0.,0.,1.));
#10951=DIRECTION('center_axis',(0.,0.,-1.));
#10952=DIRECTION('ref_axis',(1.,0.,0.));
#10953=DIRECTION('center_axis',(0.,0.,1.));
#10954=DIRECTION('ref_axis',(1.,0.,0.));
#10955=DIRECTION('center_axis',(0.,0.,1.));
#10956=DIRECTION('ref_axis',(-1.,-3.21624529935327E-16,0.));
#10957=DIRECTION('center_axis',(0.,0.,-1.));
#10958=DIRECTION('ref_axis',(1.,0.,0.));
#10959=DIRECTION('center_axis',(0.,0.,1.));
#10960=DIRECTION('ref_axis',(1.,0.,0.));
#10961=DIRECTION('center_axis',(0.,0.,1.));
#10962=DIRECTION('ref_axis',(1.,0.,0.));
#10963=DIRECTION('center_axis',(0.,1.,0.));
#10964=DIRECTION('ref_axis',(-1.,0.,0.));
#10965=DIRECTION('',(0.,0.,1.));
#10966=DIRECTION('',(-1.,0.,0.));
#10967=DIRECTION('',(0.,0.,1.));
#10968=DIRECTION('center_axis',(1.,0.,0.));
#10969=DIRECTION('ref_axis',(0.,1.,0.));
#10970=DIRECTION('',(0.,1.,0.));
#10971=DIRECTION('',(0.,0.,1.));
#10972=DIRECTION('center_axis',(0.,-1.,0.));
#10973=DIRECTION('ref_axis',(1.,0.,0.));
#10974=DIRECTION('',(1.,0.,0.));
#10975=DIRECTION('',(0.,0.,1.));
#10976=DIRECTION('center_axis',(-1.,0.,0.));
#10977=DIRECTION('ref_axis',(0.,-1.,0.));
#10978=DIRECTION('',(0.,-1.,0.));
#10979=DIRECTION('center_axis',(0.,0.,1.));
#10980=DIRECTION('ref_axis',(1.,0.,0.));
#13875=CARTESIAN_POINT('',(0.,0.,0.));
#13876=CARTESIAN_POINT('Origin',(8.77091003018116,1.,-1.3));
#13877=CARTESIAN_POINT('',(8.77091003018116,0.775,-1.2));
#13878=CARTESIAN_POINT('',(8.77091003018116,0.775,0.));
#13879=CARTESIAN_POINT('',(8.77091003018116,0.775,-1.3));
#13880=CARTESIAN_POINT('',(8.77091003018116,1.225,-1.2));
#13881=CARTESIAN_POINT('Origin',(8.77091003018116,1.,-1.2));
#13882=CARTESIAN_POINT('',(8.77091003018116,1.225,0.));
#13883=CARTESIAN_POINT('',(8.77091003018116,1.225,-1.3));
#13884=CARTESIAN_POINT('Origin',(8.77091003018116,1.,0.));
#13885=CARTESIAN_POINT('Origin',(10.7709100301812,1.,-1.3));
#13886=CARTESIAN_POINT('',(10.7709100301812,0.775,-1.2));
#13887=CARTESIAN_POINT('',(10.7709100301812,0.775,0.));
#13888=CARTESIAN_POINT('',(10.7709100301812,0.775,-1.3));
#13889=CARTESIAN_POINT('',(10.7709100301812,1.225,0.));
#13890=CARTESIAN_POINT('Origin',(10.7709100301812,1.,0.));
#13891=CARTESIAN_POINT('',(10.7709100301812,1.225,-1.2));
#13892=CARTESIAN_POINT('',(10.7709100301812,1.225,-1.3));
#13893=CARTESIAN_POINT('Origin',(10.7709100301812,1.,-1.2));
#13894=CARTESIAN_POINT('Origin',(4.,-1.,-1.2));
#13895=CARTESIAN_POINT('',(-4.,4.5,-1.2));
#13896=CARTESIAN_POINT('',(-4.,-6.5,-1.2));
#13897=CARTESIAN_POINT('',(-4.,4.5,-1.2));
#13898=CARTESIAN_POINT('',(12.,4.5,-1.2));
#13899=CARTESIAN_POINT('',(12.,4.5,-1.2));
#13900=CARTESIAN_POINT('',(12.,-6.5,-1.2));
#13901=CARTESIAN_POINT('',(12.,-6.5,-1.2));
#13902=CARTESIAN_POINT('',(-4.,-6.5,-1.2));
#13903=CARTESIAN_POINT('',(8.77091003018116,-0.775,-1.2));
#13904=CARTESIAN_POINT('',(8.77091003018116,-1.225,-1.2));
#13905=CARTESIAN_POINT('Origin',(8.77091003018116,-1.,-1.2));
#13906=CARTESIAN_POINT('',(10.7709100301812,-1.225,-1.2));
#13907=CARTESIAN_POINT('',(6.38545501509058,-1.225,-1.2));
#13908=CARTESIAN_POINT('',(10.7709100301812,-0.775,-1.2));
#13909=CARTESIAN_POINT('Origin',(10.7709100301812,-1.,-1.2));
#13910=CARTESIAN_POINT('',(7.38545501509058,-0.775,-1.2));
#13911=CARTESIAN_POINT('',(3.17091003018116,-0.775,-1.2));
#13912=CARTESIAN_POINT('',(3.17091003018116,-1.225,-1.2));
#13913=CARTESIAN_POINT('Origin',(3.17091003018116,-1.,-1.2));
#13914=CARTESIAN_POINT('',(5.17091003018116,-1.225,-1.2));
#13915=CARTESIAN_POINT('',(3.58545501509058,-1.225,-1.2));
#13916=CARTESIAN_POINT('',(5.17091003018116,-0.775,-1.2));
#13917=CARTESIAN_POINT('Origin',(5.17091003018116,-1.,-1.2));
#13918=CARTESIAN_POINT('',(4.58545501509058,-0.775,-1.2));
#13919=CARTESIAN_POINT('',(3.17091003018116,1.225,-1.2));
#13920=CARTESIAN_POINT('',(3.17091003018116,0.775,-1.2));
#13921=CARTESIAN_POINT('Origin',(3.17091003018116,1.,-1.2));
#13922=CARTESIAN_POINT('',(5.17091003018116,0.775,-1.2));
#13923=CARTESIAN_POINT('',(3.58545501509058,0.775,-1.2));
#13924=CARTESIAN_POINT('',(5.17091003018116,1.225,-1.2));
#13925=CARTESIAN_POINT('Origin',(5.17091003018116,1.,-1.2));
#13926=CARTESIAN_POINT('',(4.58545501509058,1.225,-1.2));
#13927=CARTESIAN_POINT('',(6.38545501509058,0.775,-1.2));
#13928=CARTESIAN_POINT('',(7.38545501509058,1.225,-1.2));
#13929=CARTESIAN_POINT('Origin',(10.7709100301812,1.225,-1.3));
#13930=CARTESIAN_POINT('',(7.38545501509058,1.225,0.));
#13931=CARTESIAN_POINT('Origin',(8.77091003018116,0.775,-1.3));
#13932=CARTESIAN_POINT('',(6.38545501509058,0.775,0.));
#13933=CARTESIAN_POINT('Origin',(8.77091003018116,-1.,-1.3));
#13934=CARTESIAN_POINT('',(8.77091003018116,-1.225,0.));
#13935=CARTESIAN_POINT('',(8.77091003018116,-1.225,-1.3));
#13936=CARTESIAN_POINT('',(8.77091003018116,-0.775,0.));
#13937=CARTESIAN_POINT('',(8.77091003018116,-0.775,-1.3));
#13938=CARTESIAN_POINT('Origin',(8.77091003018116,-1.,0.));
#13939=CARTESIAN_POINT('Origin',(10.7709100301812,-1.,-1.3));
#13940=CARTESIAN_POINT('',(10.7709100301812,-1.225,0.));
#13941=CARTESIAN_POINT('',(10.7709100301812,-1.225,-1.3));
#13942=CARTESIAN_POINT('',(10.7709100301812,-0.775,0.));
#13943=CARTESIAN_POINT('Origin',(10.7709100301812,-1.,0.));
#13944=CARTESIAN_POINT('',(10.7709100301812,-0.775,-1.3));
#13945=CARTESIAN_POINT('Origin',(10.7709100301812,-0.775,-1.3));
#13946=CARTESIAN_POINT('',(7.38545501509058,-0.775,0.));
#13947=CARTESIAN_POINT('Origin',(8.77091003018116,-1.225,-1.3));
#13948=CARTESIAN_POINT('',(6.38545501509058,-1.225,0.));
#13949=CARTESIAN_POINT('Origin',(3.17091003018116,1.,-1.3));
#13950=CARTESIAN_POINT('',(2.9539109773241,0.940532268757414,0.));
#13951=CARTESIAN_POINT('',(2.9539109773241,0.940532268757414,-1.1));
#13952=CARTESIAN_POINT('',(2.9539109773241,0.940532268757414,-1.3));
#13953=CARTESIAN_POINT('',(3.17091003018116,0.775,0.));
#13954=CARTESIAN_POINT('Origin',(3.17091003018116,1.,0.));
#13955=CARTESIAN_POINT('',(3.17091003018116,0.775,-1.3));
#13956=CARTESIAN_POINT('',(3.17091003018116,1.225,0.));
#13957=CARTESIAN_POINT('',(3.17091003018116,1.225,-1.3));
#13958=CARTESIAN_POINT('',(2.9539109773241,1.05946773124259,0.));
#13959=CARTESIAN_POINT('Origin',(3.17091003018116,1.,0.));
#13960=CARTESIAN_POINT('',(2.9539109773241,1.05946773124259,-1.1));
#13961=CARTESIAN_POINT('',(2.9539109773241,1.05946773124259,-1.3));
#13962=CARTESIAN_POINT('Origin',(3.17091003018116,1.,-1.1));
#13963=CARTESIAN_POINT('Origin',(5.17091003018116,1.,-1.3));
#13964=CARTESIAN_POINT('',(5.17091003018116,0.775,0.));
#13965=CARTESIAN_POINT('',(5.17091003018116,0.775,-1.3));
#13966=CARTESIAN_POINT('',(5.17091003018116,1.225,0.));
#13967=CARTESIAN_POINT('Origin',(5.17091003018116,1.,0.));
#13968=CARTESIAN_POINT('',(5.17091003018116,1.225,-1.3));
#13969=CARTESIAN_POINT('Origin',(5.17091003018116,1.225,-1.3));
#13970=CARTESIAN_POINT('',(4.58545501509058,1.225,0.));
#13971=CARTESIAN_POINT('Origin',(3.17091003018116,0.775,-1.3));
#13972=CARTESIAN_POINT('',(3.58545501509058,0.775,0.));
#13973=CARTESIAN_POINT('Origin',(3.17091003018116,-1.,-1.3));
#13974=CARTESIAN_POINT('',(2.9539109773241,-1.05946773124259,0.));
#13975=CARTESIAN_POINT('',(2.9539109773241,-1.05946773124259,-1.1));
#13976=CARTESIAN_POINT('',(2.9539109773241,-1.05946773124259,-1.3));
#13977=CARTESIAN_POINT('',(3.17091003018116,-1.225,0.));
#13978=CARTESIAN_POINT('Origin',(3.17091003018116,-1.,0.));
#13979=CARTESIAN_POINT('',(3.17091003018116,-1.225,-1.3));
#13980=CARTESIAN_POINT('',(3.17091003018116,-0.775,0.));
#13981=CARTESIAN_POINT('',(3.17091003018116,-0.775,-1.3));
#13982=CARTESIAN_POINT('',(2.9539109773241,-0.940532268757414,0.));
#13983=CARTESIAN_POINT('Origin',(3.17091003018116,-1.,0.));
#13984=CARTESIAN_POINT('',(2.9539109773241,-0.940532268757414,-1.1));
#13985=CARTESIAN_POINT('',(2.9539109773241,-0.940532268757414,-1.3));
#13986=CARTESIAN_POINT('Origin',(3.17091003018116,-1.,-1.1));
#13987=CARTESIAN_POINT('Origin',(5.17091003018116,-1.,-1.3));
#13988=CARTESIAN_POINT('',(5.17091003018116,-1.225,0.));
#13989=CARTESIAN_POINT('',(5.17091003018116,-1.225,-1.3));
#13990=CARTESIAN_POINT('',(5.17091003018116,-0.775,0.));
#13991=CARTESIAN_POINT('Origin',(5.17091003018116,-1.,0.));
#13992=CARTESIAN_POINT('',(5.17091003018116,-0.775,-1.3));
#13993=CARTESIAN_POINT('Origin',(5.17091003018116,-0.775,-1.3));
#13994=CARTESIAN_POINT('',(4.58545501509058,-0.775,0.));
#13995=CARTESIAN_POINT('Origin',(3.17091003018116,-1.225,-1.3));
#13996=CARTESIAN_POINT('',(3.58545501509058,-1.225,0.));
#13997=CARTESIAN_POINT('Origin',(2.8,-1.,-1.1));
#13998=CARTESIAN_POINT('Origin',(2.8,-1.,0.));
#13999=CARTESIAN_POINT('Origin',(2.8,-1.,-1.1));
#14000=CARTESIAN_POINT('Origin',(2.8,-1.,-1.1));
#14001=CARTESIAN_POINT('Origin',(-2.8,1.,-1.1));
#14002=CARTESIAN_POINT('',(-2.965,1.,-1.1));
#14003=CARTESIAN_POINT('Origin',(-2.8,1.,-1.1));
#14004=CARTESIAN_POINT('',(-2.965,1.,0.));
#14005=CARTESIAN_POINT('',(-2.965,1.,-1.1));
#14006=CARTESIAN_POINT('Origin',(-2.8,1.,0.));
#14007=CARTESIAN_POINT('Origin',(-2.8,1.,-1.1));
#14008=CARTESIAN_POINT('Origin',(-2.8,-1.,-1.1));
#14009=CARTESIAN_POINT('',(-2.965,-1.,-1.1));
#14010=CARTESIAN_POINT('Origin',(-2.8,-1.,-1.1));
#14011=CARTESIAN_POINT('',(-2.965,-1.,0.));
#14012=CARTESIAN_POINT('',(-2.965,-1.,-1.1));
#14013=CARTESIAN_POINT('Origin',(-2.8,-1.,0.));
#14014=CARTESIAN_POINT('Origin',(-2.8,-1.,-1.1));
#14015=CARTESIAN_POINT('Origin',(2.8,1.,-1.1));
#14016=CARTESIAN_POINT('Origin',(2.8,1.,0.));
#14017=CARTESIAN_POINT('Origin',(2.8,1.,-1.1));
#14018=CARTESIAN_POINT('Origin',(2.8,1.,-1.1));
#14019=CARTESIAN_POINT('Origin',(12.,4.5,-1.2));
#14020=CARTESIAN_POINT('',(-4.,4.5,0.));
#14021=CARTESIAN_POINT('',(-4.,4.5,-1.2));
#14022=CARTESIAN_POINT('',(12.,4.5,0.));
#14023=CARTESIAN_POINT('',(12.,4.5,0.));
#14024=CARTESIAN_POINT('',(12.,4.5,-1.2));
#14025=CARTESIAN_POINT('Origin',(12.,-6.5,-1.2));
#14026=CARTESIAN_POINT('',(12.,-6.5,0.));
#14027=CARTESIAN_POINT('',(12.,-6.5,0.));
#14028=CARTESIAN_POINT('',(12.,-6.5,-1.2));
#14029=CARTESIAN_POINT('Origin',(-4.,-6.5,-1.2));
#14030=CARTESIAN_POINT('',(-4.,-6.5,0.));
#14031=CARTESIAN_POINT('',(-4.,-6.5,0.));
#14032=CARTESIAN_POINT('',(-4.,-6.5,-1.2));
#14033=CARTESIAN_POINT('Origin',(-4.,4.5,-1.2));
#14034=CARTESIAN_POINT('',(-4.,4.5,0.));
#14035=CARTESIAN_POINT('Origin',(4.,-1.,0.));
#17733=UNCERTAINTY_MEASURE_WITH_UNIT(LENGTH_MEASURE(0.001),#17831,
'DISTANCE_ACCURACY_VALUE',
'Maximum model space distance between geometric entities at asserted c
onnectivities');
#17780=UNCERTAINTY_MEASURE_WITH_UNIT(LENGTH_MEASURE(0.001),#17831,
'DISTANCE_ACCURACY_VALUE',
'Maximum model space distance between geometric entities at asserted c
onnectivities');
#17783=(
GEOMETRIC_REPRESENTATION_CONTEXT(3)
GLOBAL_UNCERTAINTY_ASSIGNED_CONTEXT((#17733))
GLOBAL_UNIT_ASSIGNED_CONTEXT((#17831,#17833,#17834))
REPRESENTATION_CONTEXT('','3D')
);
#17830=(
GEOMETRIC_REPRESENTATION_CONTEXT(3)
GLOBAL_UNCERTAINTY_ASSIGNED_CONTEXT((#17780))
GLOBAL_UNIT_ASSIGNED_CONTEXT((#17831,#17833,#17834))
REPRESENTATION_CONTEXT('','3D')
);
#17831=(
LENGTH_UNIT()
NAMED_UNIT(*)
SI_UNIT(.CENTI.,.METRE.)
);
#17833=(
NAMED_UNIT(*)
PLANE_ANGLE_UNIT()
SI_UNIT($,.RADIAN.)
);
#17834=(
NAMED_UNIT(*)
SI_UNIT($,.STERADIAN.)
SOLID_ANGLE_UNIT()
);
#17837=SHAPE_DEFINITION_REPRESENTATION(#17886,#18008);
#17886=PRODUCT_DEFINITION_SHAPE('',$,#18058);
#18008=SHAPE_REPRESENTATION('',(#9518),#17783);
#18055=PRODUCT_DEFINITION_CONTEXT('part definition',#18204,'design');
#18058=PRODUCT_DEFINITION('Base','Base',#18107,#18055);
#18107=PRODUCT_DEFINITION_FORMATION('',$,#18208);
#18204=APPLICATION_CONTEXT(
'Core Data for Automotive Mechanical Design Process');
#18205=PRODUCT_CONTEXT('part definition',#18204,'mechanical');
#18208=PRODUCT('Base','Base','Base',(#18205));
#18290=COLOUR_RGB('Dark Blue',0.08,0.2,0.34);
#18291=FILL_AREA_STYLE_COLOUR('',#18290);
#18292=FILL_AREA_STYLE('',(#18291));
#18293=SURFACE_STYLE_FILL_AREA(#18292);
#18294=SURFACE_SIDE_STYLE('',(#18293));
#18295=SURFACE_STYLE_USAGE(.BOTH.,#18294);
#18296=PRESENTATION_STYLE_ASSIGNMENT((#18295));
ENDSEC;
END-ISO-10303-21;
